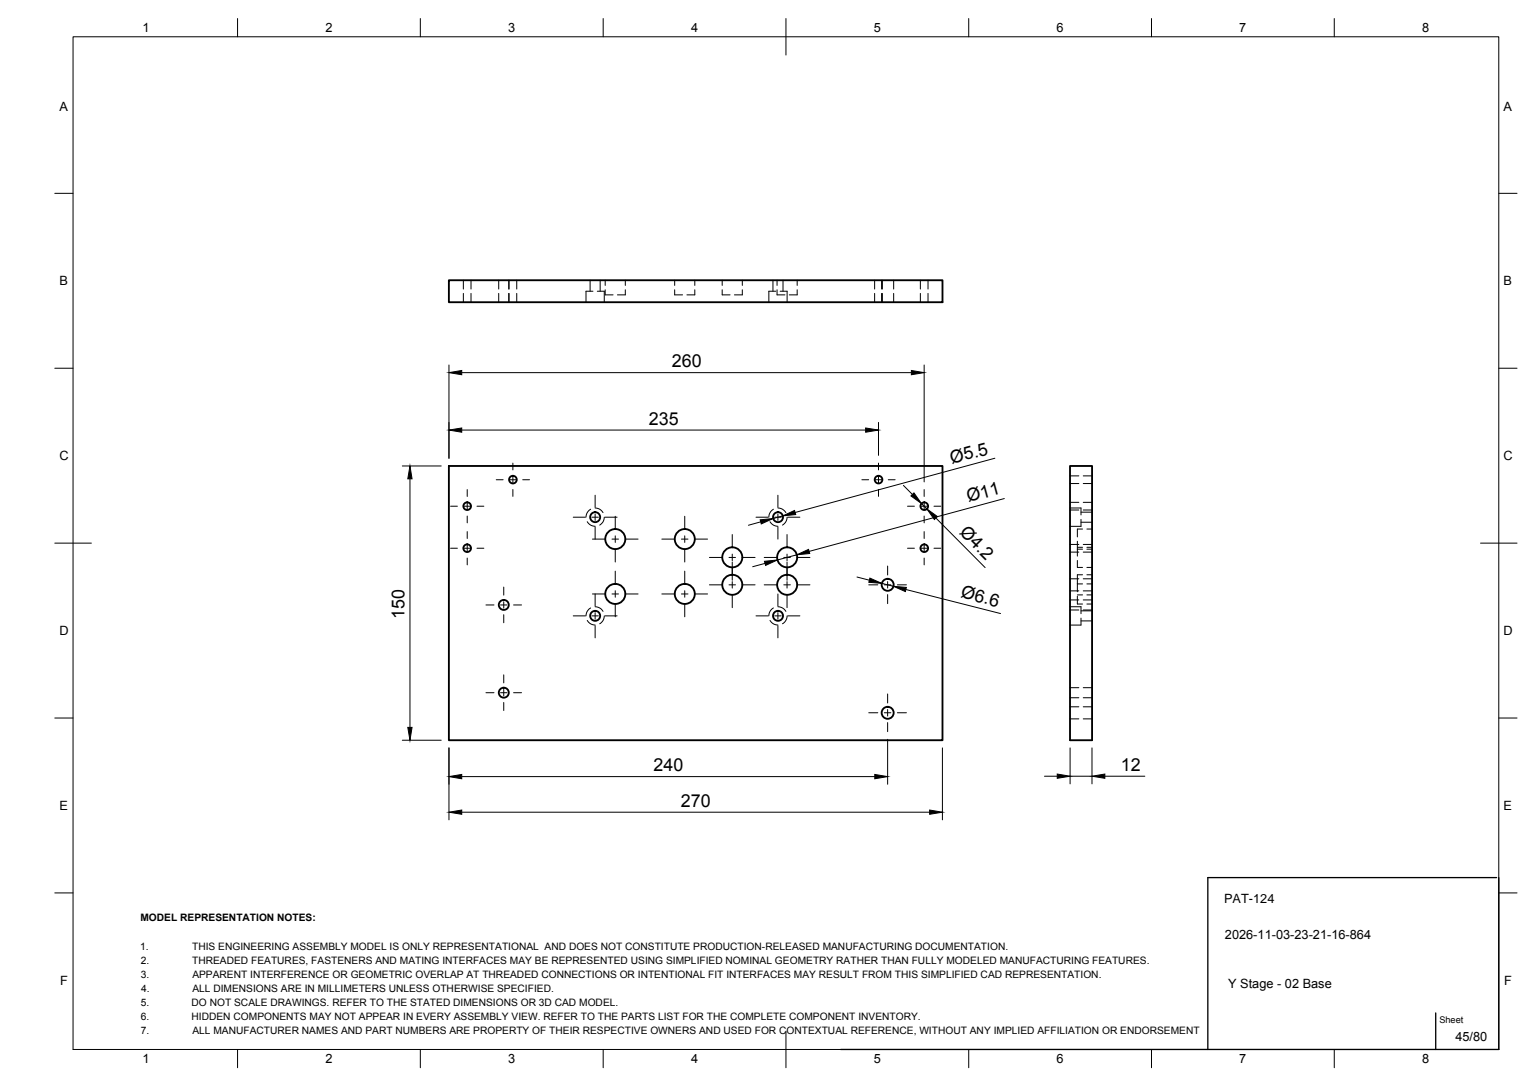
ISO-10303-21;
HEADER;
/* Generated by software containing ST-Developer
 * from STEP Tools, Inc. (www.steptools.com) 
 */

FILE_DESCRIPTION(
/* description */ ('XY cross-slide table'),
/* implementation_level */ '2;1');

FILE_NAME(
/* name */ 'Y Stage - 02 Base.step',
/* time_stamp */ '2026-10-28T03:22:46-07:00',
/* author */ (''),
/* organization */ (''),
/* preprocessor_version */ 'ST-DEVELOPER v20.2',
/* originating_system */ 'Autodesk Translation Framework v15.17.0.0',
/* authorisation */ '');

FILE_SCHEMA (('AUTOMOTIVE_DESIGN { 1 0 10303 214 3 1 1 }'));
ENDSEC;

DATA;
#10=MECHANICAL_DESIGN_GEOMETRIC_PRESENTATION_REPRESENTATION('',(#1727),#62984);
#1546=SHAPE_REPRESENTATION_RELATIONSHIP('SRR','None',#63401,#1629);
#1629=ADVANCED_BREP_SHAPE_REPRESENTATION('',(#1836),#62938);
#1727=STYLED_ITEM('',(#63891),#1836);
#1836=MANIFOLD_SOLID_BREP('Body1',#23025);
#2085=FACE_BOUND('',#5042,.T.);
#2086=FACE_BOUND('',#5045,.T.);
#2087=FACE_BOUND('',#5048,.T.);
#2088=FACE_BOUND('',#5051,.T.);
#2089=FACE_BOUND('',#5071,.T.);
#2090=FACE_BOUND('',#5072,.T.);
#2091=FACE_BOUND('',#5073,.T.);
#2092=FACE_BOUND('',#5074,.T.);
#2093=FACE_BOUND('',#5075,.T.);
#2094=FACE_BOUND('',#5076,.T.);
#2095=FACE_BOUND('',#5077,.T.);
#2096=FACE_BOUND('',#5078,.T.);
#2097=FACE_BOUND('',#5079,.T.);
#2098=FACE_BOUND('',#5080,.T.);
#2099=FACE_BOUND('',#5081,.T.);
#2100=FACE_BOUND('',#5082,.T.);
#2101=FACE_BOUND('',#5083,.T.);
#2102=FACE_BOUND('',#5084,.T.);
#2103=FACE_BOUND('',#5086,.T.);
#2104=FACE_BOUND('',#5087,.T.);
#2105=FACE_BOUND('',#5088,.T.);
#2106=FACE_BOUND('',#5089,.T.);
#2107=FACE_BOUND('',#5090,.T.);
#2108=FACE_BOUND('',#5091,.T.);
#2109=FACE_BOUND('',#5092,.T.);
#2110=FACE_BOUND('',#5093,.T.);
#2111=FACE_BOUND('',#5094,.T.);
#2112=FACE_BOUND('',#5095,.T.);
#2113=FACE_BOUND('',#5096,.T.);
#2114=FACE_BOUND('',#5097,.T.);
#2115=FACE_BOUND('',#5098,.T.);
#2116=FACE_BOUND('',#5099,.T.);
#2117=FACE_BOUND('',#5100,.T.);
#2118=FACE_BOUND('',#5101,.T.);
#2119=FACE_BOUND('',#5102,.T.);
#2120=FACE_BOUND('',#5103,.T.);
#2121=FACE_BOUND('',#5104,.T.);
#2122=FACE_BOUND('',#5105,.T.);
#2123=FACE_BOUND('',#5106,.T.);
#2124=FACE_BOUND('',#5107,.T.);
#2577=PLANE('',#25206);
#2578=PLANE('',#25210);
#2579=PLANE('',#25214);
#2580=PLANE('',#25218);
#2581=PLANE('',#25222);
#2582=PLANE('',#25226);
#2583=PLANE('',#25230);
#2584=PLANE('',#25234);
#2585=PLANE('',#25238);
#2586=PLANE('',#25243);
#2587=PLANE('',#25248);
#2588=PLANE('',#25253);
#2589=PLANE('',#25293);
#2590=PLANE('',#25294);
#2591=PLANE('',#25295);
#2592=PLANE('',#25296);
#2593=PLANE('',#25297);
#2594=PLANE('',#25298);
#3512=FACE_OUTER_BOUND('',#5024,.T.);
#3513=FACE_OUTER_BOUND('',#5025,.T.);
#3514=FACE_OUTER_BOUND('',#5026,.T.);
#3515=FACE_OUTER_BOUND('',#5027,.T.);
#3516=FACE_OUTER_BOUND('',#5028,.T.);
#3517=FACE_OUTER_BOUND('',#5029,.T.);
#3518=FACE_OUTER_BOUND('',#5030,.T.);
#3519=FACE_OUTER_BOUND('',#5031,.T.);
#3520=FACE_OUTER_BOUND('',#5032,.T.);
#3521=FACE_OUTER_BOUND('',#5033,.T.);
#3522=FACE_OUTER_BOUND('',#5034,.T.);
#3523=FACE_OUTER_BOUND('',#5035,.T.);
#3524=FACE_OUTER_BOUND('',#5036,.T.);
#3525=FACE_OUTER_BOUND('',#5037,.T.);
#3526=FACE_OUTER_BOUND('',#5038,.T.);
#3527=FACE_OUTER_BOUND('',#5039,.T.);
#3528=FACE_OUTER_BOUND('',#5040,.T.);
#3529=FACE_OUTER_BOUND('',#5041,.T.);
#3530=FACE_OUTER_BOUND('',#5043,.T.);
#3531=FACE_OUTER_BOUND('',#5044,.T.);
#3532=FACE_OUTER_BOUND('',#5046,.T.);
#3533=FACE_OUTER_BOUND('',#5047,.T.);
#3534=FACE_OUTER_BOUND('',#5049,.T.);
#3535=FACE_OUTER_BOUND('',#5050,.T.);
#3536=FACE_OUTER_BOUND('',#5052,.T.);
#3537=FACE_OUTER_BOUND('',#5053,.T.);
#3538=FACE_OUTER_BOUND('',#5054,.T.);
#3539=FACE_OUTER_BOUND('',#5055,.T.);
#3540=FACE_OUTER_BOUND('',#5056,.T.);
#3541=FACE_OUTER_BOUND('',#5057,.T.);
#3542=FACE_OUTER_BOUND('',#5058,.T.);
#3543=FACE_OUTER_BOUND('',#5059,.T.);
#3544=FACE_OUTER_BOUND('',#5060,.T.);
#3545=FACE_OUTER_BOUND('',#5061,.T.);
#3546=FACE_OUTER_BOUND('',#5062,.T.);
#3547=FACE_OUTER_BOUND('',#5063,.T.);
#3548=FACE_OUTER_BOUND('',#5064,.T.);
#3549=FACE_OUTER_BOUND('',#5065,.T.);
#3550=FACE_OUTER_BOUND('',#5066,.T.);
#3551=FACE_OUTER_BOUND('',#5067,.T.);
#3552=FACE_OUTER_BOUND('',#5068,.T.);
#3553=FACE_OUTER_BOUND('',#5069,.T.);
#3554=FACE_OUTER_BOUND('',#5070,.T.);
#3555=FACE_OUTER_BOUND('',#5085,.T.);
#5024=EDGE_LOOP('',(#17930,#17931,#17932,#17933));
#5025=EDGE_LOOP('',(#17934));
#5026=EDGE_LOOP('',(#17935,#17936,#17937,#17938));
#5027=EDGE_LOOP('',(#17939));
#5028=EDGE_LOOP('',(#17940,#17941,#17942,#17943));
#5029=EDGE_LOOP('',(#17944));
#5030=EDGE_LOOP('',(#17945,#17946,#17947,#17948));
#5031=EDGE_LOOP('',(#17949));
#5032=EDGE_LOOP('',(#17950,#17951,#17952,#17953));
#5033=EDGE_LOOP('',(#17954));
#5034=EDGE_LOOP('',(#17955,#17956,#17957,#17958));
#5035=EDGE_LOOP('',(#17959));
#5036=EDGE_LOOP('',(#17960,#17961,#17962,#17963));
#5037=EDGE_LOOP('',(#17964));
#5038=EDGE_LOOP('',(#17965,#17966,#17967,#17968));
#5039=EDGE_LOOP('',(#17969));
#5040=EDGE_LOOP('',(#17970,#17971,#17972,#17973));
#5041=EDGE_LOOP('',(#17974));
#5042=EDGE_LOOP('',(#17975));
#5043=EDGE_LOOP('',(#17976,#17977,#17978,#17979));
#5044=EDGE_LOOP('',(#17980));
#5045=EDGE_LOOP('',(#17981));
#5046=EDGE_LOOP('',(#17982,#17983,#17984,#17985));
#5047=EDGE_LOOP('',(#17986));
#5048=EDGE_LOOP('',(#17987));
#5049=EDGE_LOOP('',(#17988,#17989,#17990,#17991));
#5050=EDGE_LOOP('',(#17992));
#5051=EDGE_LOOP('',(#17993));
#5052=EDGE_LOOP('',(#17994,#17995,#17996,#17997));
#5053=EDGE_LOOP('',(#17998,#17999,#18000,#18001));
#5054=EDGE_LOOP('',(#18002,#18003,#18004,#18005));
#5055=EDGE_LOOP('',(#18006,#18007,#18008,#18009));
#5056=EDGE_LOOP('',(#18010,#18011,#18012,#18013));
#5057=EDGE_LOOP('',(#18014,#18015,#18016,#18017));
#5058=EDGE_LOOP('',(#18018,#18019,#18020,#18021));
#5059=EDGE_LOOP('',(#18022,#18023,#18024,#18025));
#5060=EDGE_LOOP('',(#18026,#18027,#18028,#18029));
#5061=EDGE_LOOP('',(#18030,#18031,#18032,#18033));
#5062=EDGE_LOOP('',(#18034,#18035,#18036,#18037));
#5063=EDGE_LOOP('',(#18038,#18039,#18040,#18041));
#5064=EDGE_LOOP('',(#18042,#18043,#18044,#18045));
#5065=EDGE_LOOP('',(#18046,#18047,#18048,#18049));
#5066=EDGE_LOOP('',(#18050,#18051,#18052,#18053));
#5067=EDGE_LOOP('',(#18054,#18055,#18056,#18057));
#5068=EDGE_LOOP('',(#18058,#18059,#18060,#18061));
#5069=EDGE_LOOP('',(#18062,#18063,#18064,#18065));
#5070=EDGE_LOOP('',(#18066,#18067,#18068,#18069));
#5071=EDGE_LOOP('',(#18070));
#5072=EDGE_LOOP('',(#18071));
#5073=EDGE_LOOP('',(#18072));
#5074=EDGE_LOOP('',(#18073));
#5075=EDGE_LOOP('',(#18074));
#5076=EDGE_LOOP('',(#18075));
#5077=EDGE_LOOP('',(#18076));
#5078=EDGE_LOOP('',(#18077));
#5079=EDGE_LOOP('',(#18078));
#5080=EDGE_LOOP('',(#18079));
#5081=EDGE_LOOP('',(#18080));
#5082=EDGE_LOOP('',(#18081));
#5083=EDGE_LOOP('',(#18082));
#5084=EDGE_LOOP('',(#18083));
#5085=EDGE_LOOP('',(#18084,#18085,#18086,#18087));
#5086=EDGE_LOOP('',(#18088));
#5087=EDGE_LOOP('',(#18089));
#5088=EDGE_LOOP('',(#18090));
#5089=EDGE_LOOP('',(#18091));
#5090=EDGE_LOOP('',(#18092));
#5091=EDGE_LOOP('',(#18093));
#5092=EDGE_LOOP('',(#18094));
#5093=EDGE_LOOP('',(#18095));
#5094=EDGE_LOOP('',(#18096));
#5095=EDGE_LOOP('',(#18097));
#5096=EDGE_LOOP('',(#18098));
#5097=EDGE_LOOP('',(#18099));
#5098=EDGE_LOOP('',(#18100));
#5099=EDGE_LOOP('',(#18101));
#5100=EDGE_LOOP('',(#18102));
#5101=EDGE_LOOP('',(#18103));
#5102=EDGE_LOOP('',(#18104));
#5103=EDGE_LOOP('',(#18105));
#5104=EDGE_LOOP('',(#18106));
#5105=EDGE_LOOP('',(#18107));
#5106=EDGE_LOOP('',(#18108));
#5107=EDGE_LOOP('',(#18109));
#6644=LINE('',#47786,#8131);
#6645=LINE('',#47793,#8132);
#6646=LINE('',#47800,#8133);
#6647=LINE('',#47807,#8134);
#6648=LINE('',#47814,#8135);
#6649=LINE('',#47821,#8136);
#6650=LINE('',#47828,#8137);
#6651=LINE('',#47835,#8138);
#6652=LINE('',#47842,#8139);
#6653=LINE('',#47851,#8140);
#6654=LINE('',#47860,#8141);
#6655=LINE('',#47869,#8142);
#6656=LINE('',#47877,#8143);
#6657=LINE('',#47881,#8144);
#6658=LINE('',#47885,#8145);
#6659=LINE('',#47889,#8146);
#6660=LINE('',#47894,#8147);
#6661=LINE('',#47900,#8148);
#6662=LINE('',#47906,#8149);
#6663=LINE('',#47912,#8150);
#6664=LINE('',#47918,#8151);
#6665=LINE('',#47924,#8152);
#6666=LINE('',#47930,#8153);
#6667=LINE('',#47936,#8154);
#6668=LINE('',#47942,#8155);
#6669=LINE('',#47948,#8156);
#6670=LINE('',#47953,#8157);
#6671=LINE('',#47955,#8158);
#6672=LINE('',#47957,#8159);
#6673=LINE('',#47958,#8160);
#6674=LINE('',#47961,#8161);
#6675=LINE('',#47963,#8162);
#6676=LINE('',#47964,#8163);
#6677=LINE('',#47967,#8164);
#6678=LINE('',#47969,#8165);
#6679=LINE('',#47970,#8166);
#6680=LINE('',#47972,#8167);
#6681=LINE('',#47973,#8168);
#8131=VECTOR('',#29609,0.550000000000001);
#8132=VECTOR('',#29618,0.550000000000001);
#8133=VECTOR('',#29627,0.550000000000001);
#8134=VECTOR('',#29636,0.550000000000001);
#8135=VECTOR('',#29645,0.550000000000001);
#8136=VECTOR('',#29654,0.550000000000001);
#8137=VECTOR('',#29663,0.550000000000001);
#8138=VECTOR('',#29672,0.550000000000001);
#8139=VECTOR('',#29681,0.5);
#8140=VECTOR('',#29692,0.5);
#8141=VECTOR('',#29703,0.5);
#8142=VECTOR('',#29714,0.5);
#8143=VECTOR('',#29725,0.275);
#8144=VECTOR('',#29730,0.274999999999999);
#8145=VECTOR('',#29735,0.275);
#8146=VECTOR('',#29740,0.274999999999999);
#8147=VECTOR('',#29745,0.210000000000001);
#8148=VECTOR('',#29752,0.21);
#8149=VECTOR('',#29759,0.329999999999998);
#8150=VECTOR('',#29766,0.329999999999998);
#8151=VECTOR('',#29773,0.275);
#8152=VECTOR('',#29780,0.275);
#8153=VECTOR('',#29787,0.210000000000001);
#8154=VECTOR('',#29794,0.21);
#8155=VECTOR('',#29801,0.21);
#8156=VECTOR('',#29808,0.210000000000001);
#8157=VECTOR('',#29813,1.);
#8158=VECTOR('',#29814,1.);
#8159=VECTOR('',#29815,1.);
#8160=VECTOR('',#29816,1.);
#8161=VECTOR('',#29819,1.);
#8162=VECTOR('',#29820,1.);
#8163=VECTOR('',#29821,1.);
#8164=VECTOR('',#29824,1.);
#8165=VECTOR('',#29825,1.);
#8166=VECTOR('',#29826,1.);
#8167=VECTOR('',#29829,1.);
#8168=VECTOR('',#29830,1.);
#9311=CIRCLE('',#25204,0.550000000000001);
#9312=CIRCLE('',#25205,0.550000000000001);
#9313=CIRCLE('',#25208,0.550000000000001);
#9314=CIRCLE('',#25209,0.550000000000001);
#9315=CIRCLE('',#25212,0.550000000000001);
#9316=CIRCLE('',#25213,0.550000000000001);
#9317=CIRCLE('',#25216,0.550000000000001);
#9318=CIRCLE('',#25217,0.550000000000001);
#9319=CIRCLE('',#25220,0.550000000000001);
#9320=CIRCLE('',#25221,0.550000000000001);
#9321=CIRCLE('',#25224,0.550000000000001);
#9322=CIRCLE('',#25225,0.550000000000001);
#9323=CIRCLE('',#25228,0.550000000000001);
#9324=CIRCLE('',#25229,0.550000000000001);
#9325=CIRCLE('',#25232,0.550000000000001);
#9326=CIRCLE('',#25233,0.550000000000001);
#9327=CIRCLE('',#25236,0.5);
#9328=CIRCLE('',#25237,0.5);
#9329=CIRCLE('',#25239,0.275);
#9330=CIRCLE('',#25241,0.5);
#9331=CIRCLE('',#25242,0.5);
#9332=CIRCLE('',#25244,0.274999999999999);
#9333=CIRCLE('',#25246,0.5);
#9334=CIRCLE('',#25247,0.5);
#9335=CIRCLE('',#25249,0.275);
#9336=CIRCLE('',#25251,0.5);
#9337=CIRCLE('',#25252,0.5);
#9338=CIRCLE('',#25254,0.274999999999999);
#9339=CIRCLE('',#25256,0.275);
#9340=CIRCLE('',#25258,0.274999999999999);
#9341=CIRCLE('',#25260,0.275);
#9342=CIRCLE('',#25262,0.274999999999999);
#9343=CIRCLE('',#25264,0.210000000000001);
#9344=CIRCLE('',#25265,0.210000000000001);
#9345=CIRCLE('',#25267,0.21);
#9346=CIRCLE('',#25268,0.21);
#9347=CIRCLE('',#25270,0.329999999999998);
#9348=CIRCLE('',#25271,0.329999999999998);
#9349=CIRCLE('',#25273,0.329999999999998);
#9350=CIRCLE('',#25274,0.329999999999998);
#9351=CIRCLE('',#25276,0.275);
#9352=CIRCLE('',#25277,0.275);
#9353=CIRCLE('',#25279,0.275);
#9354=CIRCLE('',#25280,0.275);
#9355=CIRCLE('',#25282,0.210000000000001);
#9356=CIRCLE('',#25283,0.210000000000001);
#9357=CIRCLE('',#25285,0.21);
#9358=CIRCLE('',#25286,0.21);
#9359=CIRCLE('',#25288,0.21);
#9360=CIRCLE('',#25289,0.21);
#9361=CIRCLE('',#25291,0.210000000000001);
#9362=CIRCLE('',#25292,0.210000000000001);
#10791=VERTEX_POINT('',#47783);
#10792=VERTEX_POINT('',#47785);
#10793=VERTEX_POINT('',#47790);
#10794=VERTEX_POINT('',#47792);
#10795=VERTEX_POINT('',#47797);
#10796=VERTEX_POINT('',#47799);
#10797=VERTEX_POINT('',#47804);
#10798=VERTEX_POINT('',#47806);
#10799=VERTEX_POINT('',#47811);
#10800=VERTEX_POINT('',#47813);
#10801=VERTEX_POINT('',#47818);
#10802=VERTEX_POINT('',#47820);
#10803=VERTEX_POINT('',#47825);
#10804=VERTEX_POINT('',#47827);
#10805=VERTEX_POINT('',#47832);
#10806=VERTEX_POINT('',#47834);
#10807=VERTEX_POINT('',#47839);
#10808=VERTEX_POINT('',#47841);
#10809=VERTEX_POINT('',#47845);
#10810=VERTEX_POINT('',#47848);
#10811=VERTEX_POINT('',#47850);
#10812=VERTEX_POINT('',#47854);
#10813=VERTEX_POINT('',#47857);
#10814=VERTEX_POINT('',#47859);
#10815=VERTEX_POINT('',#47863);
#10816=VERTEX_POINT('',#47866);
#10817=VERTEX_POINT('',#47868);
#10818=VERTEX_POINT('',#47872);
#10819=VERTEX_POINT('',#47875);
#10820=VERTEX_POINT('',#47879);
#10821=VERTEX_POINT('',#47883);
#10822=VERTEX_POINT('',#47887);
#10823=VERTEX_POINT('',#47891);
#10824=VERTEX_POINT('',#47893);
#10825=VERTEX_POINT('',#47897);
#10826=VERTEX_POINT('',#47899);
#10827=VERTEX_POINT('',#47903);
#10828=VERTEX_POINT('',#47905);
#10829=VERTEX_POINT('',#47909);
#10830=VERTEX_POINT('',#47911);
#10831=VERTEX_POINT('',#47915);
#10832=VERTEX_POINT('',#47917);
#10833=VERTEX_POINT('',#47921);
#10834=VERTEX_POINT('',#47923);
#10835=VERTEX_POINT('',#47927);
#10836=VERTEX_POINT('',#47929);
#10837=VERTEX_POINT('',#47933);
#10838=VERTEX_POINT('',#47935);
#10839=VERTEX_POINT('',#47939);
#10840=VERTEX_POINT('',#47941);
#10841=VERTEX_POINT('',#47945);
#10842=VERTEX_POINT('',#47947);
#10843=VERTEX_POINT('',#47951);
#10844=VERTEX_POINT('',#47952);
#10845=VERTEX_POINT('',#47954);
#10846=VERTEX_POINT('',#47956);
#10847=VERTEX_POINT('',#47960);
#10848=VERTEX_POINT('',#47962);
#10849=VERTEX_POINT('',#47966);
#10850=VERTEX_POINT('',#47968);
#13349=EDGE_CURVE('',#10791,#10791,#9311,.T.);
#13350=EDGE_CURVE('',#10791,#10792,#6644,.T.);
#13351=EDGE_CURVE('',#10792,#10792,#9312,.T.);
#13352=EDGE_CURVE('',#10793,#10793,#9313,.T.);
#13353=EDGE_CURVE('',#10793,#10794,#6645,.T.);
#13354=EDGE_CURVE('',#10794,#10794,#9314,.T.);
#13355=EDGE_CURVE('',#10795,#10795,#9315,.T.);
#13356=EDGE_CURVE('',#10795,#10796,#6646,.T.);
#13357=EDGE_CURVE('',#10796,#10796,#9316,.T.);
#13358=EDGE_CURVE('',#10797,#10797,#9317,.T.);
#13359=EDGE_CURVE('',#10797,#10798,#6647,.T.);
#13360=EDGE_CURVE('',#10798,#10798,#9318,.T.);
#13361=EDGE_CURVE('',#10799,#10799,#9319,.T.);
#13362=EDGE_CURVE('',#10799,#10800,#6648,.T.);
#13363=EDGE_CURVE('',#10800,#10800,#9320,.T.);
#13364=EDGE_CURVE('',#10801,#10801,#9321,.T.);
#13365=EDGE_CURVE('',#10801,#10802,#6649,.T.);
#13366=EDGE_CURVE('',#10802,#10802,#9322,.T.);
#13367=EDGE_CURVE('',#10803,#10803,#9323,.T.);
#13368=EDGE_CURVE('',#10803,#10804,#6650,.T.);
#13369=EDGE_CURVE('',#10804,#10804,#9324,.T.);
#13370=EDGE_CURVE('',#10805,#10805,#9325,.T.);
#13371=EDGE_CURVE('',#10805,#10806,#6651,.T.);
#13372=EDGE_CURVE('',#10806,#10806,#9326,.T.);
#13373=EDGE_CURVE('',#10807,#10807,#9327,.T.);
#13374=EDGE_CURVE('',#10807,#10808,#6652,.T.);
#13375=EDGE_CURVE('',#10808,#10808,#9328,.T.);
#13376=EDGE_CURVE('',#10809,#10809,#9329,.T.);
#13377=EDGE_CURVE('',#10810,#10810,#9330,.T.);
#13378=EDGE_CURVE('',#10810,#10811,#6653,.T.);
#13379=EDGE_CURVE('',#10811,#10811,#9331,.T.);
#13380=EDGE_CURVE('',#10812,#10812,#9332,.T.);
#13381=EDGE_CURVE('',#10813,#10813,#9333,.T.);
#13382=EDGE_CURVE('',#10813,#10814,#6654,.T.);
#13383=EDGE_CURVE('',#10814,#10814,#9334,.T.);
#13384=EDGE_CURVE('',#10815,#10815,#9335,.T.);
#13385=EDGE_CURVE('',#10816,#10816,#9336,.T.);
#13386=EDGE_CURVE('',#10816,#10817,#6655,.T.);
#13387=EDGE_CURVE('',#10817,#10817,#9337,.T.);
#13388=EDGE_CURVE('',#10818,#10818,#9338,.T.);
#13389=EDGE_CURVE('',#10819,#10819,#9339,.T.);
#13390=EDGE_CURVE('',#10819,#10809,#6656,.T.);
#13391=EDGE_CURVE('',#10820,#10820,#9340,.T.);
#13392=EDGE_CURVE('',#10820,#10812,#6657,.T.);
#13393=EDGE_CURVE('',#10821,#10821,#9341,.T.);
#13394=EDGE_CURVE('',#10821,#10815,#6658,.T.);
#13395=EDGE_CURVE('',#10822,#10822,#9342,.T.);
#13396=EDGE_CURVE('',#10822,#10818,#6659,.T.);
#13397=EDGE_CURVE('',#10823,#10823,#9343,.T.);
#13398=EDGE_CURVE('',#10823,#10824,#6660,.T.);
#13399=EDGE_CURVE('',#10824,#10824,#9344,.T.);
#13400=EDGE_CURVE('',#10825,#10825,#9345,.T.);
#13401=EDGE_CURVE('',#10825,#10826,#6661,.T.);
#13402=EDGE_CURVE('',#10826,#10826,#9346,.T.);
#13403=EDGE_CURVE('',#10827,#10827,#9347,.T.);
#13404=EDGE_CURVE('',#10827,#10828,#6662,.T.);
#13405=EDGE_CURVE('',#10828,#10828,#9348,.T.);
#13406=EDGE_CURVE('',#10829,#10829,#9349,.T.);
#13407=EDGE_CURVE('',#10829,#10830,#6663,.T.);
#13408=EDGE_CURVE('',#10830,#10830,#9350,.T.);
#13409=EDGE_CURVE('',#10831,#10831,#9351,.T.);
#13410=EDGE_CURVE('',#10831,#10832,#6664,.T.);
#13411=EDGE_CURVE('',#10832,#10832,#9352,.T.);
#13412=EDGE_CURVE('',#10833,#10833,#9353,.T.);
#13413=EDGE_CURVE('',#10833,#10834,#6665,.T.);
#13414=EDGE_CURVE('',#10834,#10834,#9354,.T.);
#13415=EDGE_CURVE('',#10835,#10835,#9355,.T.);
#13416=EDGE_CURVE('',#10835,#10836,#6666,.T.);
#13417=EDGE_CURVE('',#10836,#10836,#9356,.T.);
#13418=EDGE_CURVE('',#10837,#10837,#9357,.T.);
#13419=EDGE_CURVE('',#10837,#10838,#6667,.T.);
#13420=EDGE_CURVE('',#10838,#10838,#9358,.T.);
#13421=EDGE_CURVE('',#10839,#10839,#9359,.T.);
#13422=EDGE_CURVE('',#10839,#10840,#6668,.T.);
#13423=EDGE_CURVE('',#10840,#10840,#9360,.T.);
#13424=EDGE_CURVE('',#10841,#10841,#9361,.T.);
#13425=EDGE_CURVE('',#10841,#10842,#6669,.T.);
#13426=EDGE_CURVE('',#10842,#10842,#9362,.T.);
#13427=EDGE_CURVE('',#10843,#10844,#6670,.T.);
#13428=EDGE_CURVE('',#10844,#10845,#6671,.T.);
#13429=EDGE_CURVE('',#10846,#10845,#6672,.T.);
#13430=EDGE_CURVE('',#10843,#10846,#6673,.T.);
#13431=EDGE_CURVE('',#10847,#10843,#6674,.T.);
#13432=EDGE_CURVE('',#10848,#10846,#6675,.T.);
#13433=EDGE_CURVE('',#10847,#10848,#6676,.T.);
#13434=EDGE_CURVE('',#10849,#10847,#6677,.T.);
#13435=EDGE_CURVE('',#10850,#10848,#6678,.T.);
#13436=EDGE_CURVE('',#10849,#10850,#6679,.T.);
#13437=EDGE_CURVE('',#10844,#10849,#6680,.T.);
#13438=EDGE_CURVE('',#10845,#10850,#6681,.T.);
#17930=ORIENTED_EDGE('',*,*,#13349,.F.);
#17931=ORIENTED_EDGE('',*,*,#13350,.T.);
#17932=ORIENTED_EDGE('',*,*,#13351,.T.);
#17933=ORIENTED_EDGE('',*,*,#13350,.F.);
#17934=ORIENTED_EDGE('',*,*,#13351,.F.);
#17935=ORIENTED_EDGE('',*,*,#13352,.F.);
#17936=ORIENTED_EDGE('',*,*,#13353,.T.);
#17937=ORIENTED_EDGE('',*,*,#13354,.T.);
#17938=ORIENTED_EDGE('',*,*,#13353,.F.);
#17939=ORIENTED_EDGE('',*,*,#13354,.F.);
#17940=ORIENTED_EDGE('',*,*,#13355,.F.);
#17941=ORIENTED_EDGE('',*,*,#13356,.T.);
#17942=ORIENTED_EDGE('',*,*,#13357,.T.);
#17943=ORIENTED_EDGE('',*,*,#13356,.F.);
#17944=ORIENTED_EDGE('',*,*,#13357,.F.);
#17945=ORIENTED_EDGE('',*,*,#13358,.F.);
#17946=ORIENTED_EDGE('',*,*,#13359,.T.);
#17947=ORIENTED_EDGE('',*,*,#13360,.T.);
#17948=ORIENTED_EDGE('',*,*,#13359,.F.);
#17949=ORIENTED_EDGE('',*,*,#13360,.F.);
#17950=ORIENTED_EDGE('',*,*,#13361,.F.);
#17951=ORIENTED_EDGE('',*,*,#13362,.T.);
#17952=ORIENTED_EDGE('',*,*,#13363,.T.);
#17953=ORIENTED_EDGE('',*,*,#13362,.F.);
#17954=ORIENTED_EDGE('',*,*,#13363,.F.);
#17955=ORIENTED_EDGE('',*,*,#13364,.F.);
#17956=ORIENTED_EDGE('',*,*,#13365,.T.);
#17957=ORIENTED_EDGE('',*,*,#13366,.T.);
#17958=ORIENTED_EDGE('',*,*,#13365,.F.);
#17959=ORIENTED_EDGE('',*,*,#13366,.F.);
#17960=ORIENTED_EDGE('',*,*,#13367,.F.);
#17961=ORIENTED_EDGE('',*,*,#13368,.T.);
#17962=ORIENTED_EDGE('',*,*,#13369,.T.);
#17963=ORIENTED_EDGE('',*,*,#13368,.F.);
#17964=ORIENTED_EDGE('',*,*,#13369,.F.);
#17965=ORIENTED_EDGE('',*,*,#13370,.F.);
#17966=ORIENTED_EDGE('',*,*,#13371,.T.);
#17967=ORIENTED_EDGE('',*,*,#13372,.T.);
#17968=ORIENTED_EDGE('',*,*,#13371,.F.);
#17969=ORIENTED_EDGE('',*,*,#13372,.F.);
#17970=ORIENTED_EDGE('',*,*,#13373,.F.);
#17971=ORIENTED_EDGE('',*,*,#13374,.T.);
#17972=ORIENTED_EDGE('',*,*,#13375,.F.);
#17973=ORIENTED_EDGE('',*,*,#13374,.F.);
#17974=ORIENTED_EDGE('',*,*,#13373,.T.);
#17975=ORIENTED_EDGE('',*,*,#13376,.F.);
#17976=ORIENTED_EDGE('',*,*,#13377,.F.);
#17977=ORIENTED_EDGE('',*,*,#13378,.T.);
#17978=ORIENTED_EDGE('',*,*,#13379,.F.);
#17979=ORIENTED_EDGE('',*,*,#13378,.F.);
#17980=ORIENTED_EDGE('',*,*,#13377,.T.);
#17981=ORIENTED_EDGE('',*,*,#13380,.F.);
#17982=ORIENTED_EDGE('',*,*,#13381,.F.);
#17983=ORIENTED_EDGE('',*,*,#13382,.T.);
#17984=ORIENTED_EDGE('',*,*,#13383,.F.);
#17985=ORIENTED_EDGE('',*,*,#13382,.F.);
#17986=ORIENTED_EDGE('',*,*,#13381,.T.);
#17987=ORIENTED_EDGE('',*,*,#13384,.F.);
#17988=ORIENTED_EDGE('',*,*,#13385,.F.);
#17989=ORIENTED_EDGE('',*,*,#13386,.T.);
#17990=ORIENTED_EDGE('',*,*,#13387,.F.);
#17991=ORIENTED_EDGE('',*,*,#13386,.F.);
#17992=ORIENTED_EDGE('',*,*,#13385,.T.);
#17993=ORIENTED_EDGE('',*,*,#13388,.F.);
#17994=ORIENTED_EDGE('',*,*,#13389,.F.);
#17995=ORIENTED_EDGE('',*,*,#13390,.T.);
#17996=ORIENTED_EDGE('',*,*,#13376,.T.);
#17997=ORIENTED_EDGE('',*,*,#13390,.F.);
#17998=ORIENTED_EDGE('',*,*,#13391,.F.);
#17999=ORIENTED_EDGE('',*,*,#13392,.T.);
#18000=ORIENTED_EDGE('',*,*,#13380,.T.);
#18001=ORIENTED_EDGE('',*,*,#13392,.F.);
#18002=ORIENTED_EDGE('',*,*,#13393,.F.);
#18003=ORIENTED_EDGE('',*,*,#13394,.T.);
#18004=ORIENTED_EDGE('',*,*,#13384,.T.);
#18005=ORIENTED_EDGE('',*,*,#13394,.F.);
#18006=ORIENTED_EDGE('',*,*,#13395,.F.);
#18007=ORIENTED_EDGE('',*,*,#13396,.T.);
#18008=ORIENTED_EDGE('',*,*,#13388,.T.);
#18009=ORIENTED_EDGE('',*,*,#13396,.F.);
#18010=ORIENTED_EDGE('',*,*,#13397,.F.);
#18011=ORIENTED_EDGE('',*,*,#13398,.T.);
#18012=ORIENTED_EDGE('',*,*,#13399,.F.);
#18013=ORIENTED_EDGE('',*,*,#13398,.F.);
#18014=ORIENTED_EDGE('',*,*,#13400,.F.);
#18015=ORIENTED_EDGE('',*,*,#13401,.T.);
#18016=ORIENTED_EDGE('',*,*,#13402,.F.);
#18017=ORIENTED_EDGE('',*,*,#13401,.F.);
#18018=ORIENTED_EDGE('',*,*,#13403,.F.);
#18019=ORIENTED_EDGE('',*,*,#13404,.T.);
#18020=ORIENTED_EDGE('',*,*,#13405,.F.);
#18021=ORIENTED_EDGE('',*,*,#13404,.F.);
#18022=ORIENTED_EDGE('',*,*,#13406,.F.);
#18023=ORIENTED_EDGE('',*,*,#13407,.T.);
#18024=ORIENTED_EDGE('',*,*,#13408,.F.);
#18025=ORIENTED_EDGE('',*,*,#13407,.F.);
#18026=ORIENTED_EDGE('',*,*,#13409,.F.);
#18027=ORIENTED_EDGE('',*,*,#13410,.T.);
#18028=ORIENTED_EDGE('',*,*,#13411,.F.);
#18029=ORIENTED_EDGE('',*,*,#13410,.F.);
#18030=ORIENTED_EDGE('',*,*,#13412,.F.);
#18031=ORIENTED_EDGE('',*,*,#13413,.T.);
#18032=ORIENTED_EDGE('',*,*,#13414,.F.);
#18033=ORIENTED_EDGE('',*,*,#13413,.F.);
#18034=ORIENTED_EDGE('',*,*,#13415,.F.);
#18035=ORIENTED_EDGE('',*,*,#13416,.T.);
#18036=ORIENTED_EDGE('',*,*,#13417,.F.);
#18037=ORIENTED_EDGE('',*,*,#13416,.F.);
#18038=ORIENTED_EDGE('',*,*,#13418,.F.);
#18039=ORIENTED_EDGE('',*,*,#13419,.T.);
#18040=ORIENTED_EDGE('',*,*,#13420,.F.);
#18041=ORIENTED_EDGE('',*,*,#13419,.F.);
#18042=ORIENTED_EDGE('',*,*,#13421,.F.);
#18043=ORIENTED_EDGE('',*,*,#13422,.T.);
#18044=ORIENTED_EDGE('',*,*,#13423,.F.);
#18045=ORIENTED_EDGE('',*,*,#13422,.F.);
#18046=ORIENTED_EDGE('',*,*,#13424,.F.);
#18047=ORIENTED_EDGE('',*,*,#13425,.T.);
#18048=ORIENTED_EDGE('',*,*,#13426,.F.);
#18049=ORIENTED_EDGE('',*,*,#13425,.F.);
#18050=ORIENTED_EDGE('',*,*,#13427,.T.);
#18051=ORIENTED_EDGE('',*,*,#13428,.T.);
#18052=ORIENTED_EDGE('',*,*,#13429,.F.);
#18053=ORIENTED_EDGE('',*,*,#13430,.F.);
#18054=ORIENTED_EDGE('',*,*,#13431,.T.);
#18055=ORIENTED_EDGE('',*,*,#13430,.T.);
#18056=ORIENTED_EDGE('',*,*,#13432,.F.);
#18057=ORIENTED_EDGE('',*,*,#13433,.F.);
#18058=ORIENTED_EDGE('',*,*,#13434,.T.);
#18059=ORIENTED_EDGE('',*,*,#13433,.T.);
#18060=ORIENTED_EDGE('',*,*,#13435,.F.);
#18061=ORIENTED_EDGE('',*,*,#13436,.F.);
#18062=ORIENTED_EDGE('',*,*,#13437,.T.);
#18063=ORIENTED_EDGE('',*,*,#13436,.T.);
#18064=ORIENTED_EDGE('',*,*,#13438,.F.);
#18065=ORIENTED_EDGE('',*,*,#13428,.F.);
#18066=ORIENTED_EDGE('',*,*,#13438,.T.);
#18067=ORIENTED_EDGE('',*,*,#13435,.T.);
#18068=ORIENTED_EDGE('',*,*,#13432,.T.);
#18069=ORIENTED_EDGE('',*,*,#13429,.T.);
#18070=ORIENTED_EDGE('',*,*,#13402,.T.);
#18071=ORIENTED_EDGE('',*,*,#13426,.T.);
#18072=ORIENTED_EDGE('',*,*,#13423,.T.);
#18073=ORIENTED_EDGE('',*,*,#13420,.T.);
#18074=ORIENTED_EDGE('',*,*,#13417,.T.);
#18075=ORIENTED_EDGE('',*,*,#13414,.T.);
#18076=ORIENTED_EDGE('',*,*,#13411,.T.);
#18077=ORIENTED_EDGE('',*,*,#13408,.T.);
#18078=ORIENTED_EDGE('',*,*,#13405,.T.);
#18079=ORIENTED_EDGE('',*,*,#13399,.T.);
#18080=ORIENTED_EDGE('',*,*,#13387,.T.);
#18081=ORIENTED_EDGE('',*,*,#13383,.T.);
#18082=ORIENTED_EDGE('',*,*,#13379,.T.);
#18083=ORIENTED_EDGE('',*,*,#13375,.T.);
#18084=ORIENTED_EDGE('',*,*,#13437,.F.);
#18085=ORIENTED_EDGE('',*,*,#13427,.F.);
#18086=ORIENTED_EDGE('',*,*,#13431,.F.);
#18087=ORIENTED_EDGE('',*,*,#13434,.F.);
#18088=ORIENTED_EDGE('',*,*,#13389,.T.);
#18089=ORIENTED_EDGE('',*,*,#13391,.T.);
#18090=ORIENTED_EDGE('',*,*,#13393,.T.);
#18091=ORIENTED_EDGE('',*,*,#13395,.T.);
#18092=ORIENTED_EDGE('',*,*,#13400,.T.);
#18093=ORIENTED_EDGE('',*,*,#13424,.T.);
#18094=ORIENTED_EDGE('',*,*,#13421,.T.);
#18095=ORIENTED_EDGE('',*,*,#13418,.T.);
#18096=ORIENTED_EDGE('',*,*,#13415,.T.);
#18097=ORIENTED_EDGE('',*,*,#13412,.T.);
#18098=ORIENTED_EDGE('',*,*,#13409,.T.);
#18099=ORIENTED_EDGE('',*,*,#13406,.T.);
#18100=ORIENTED_EDGE('',*,*,#13403,.T.);
#18101=ORIENTED_EDGE('',*,*,#13397,.T.);
#18102=ORIENTED_EDGE('',*,*,#13370,.T.);
#18103=ORIENTED_EDGE('',*,*,#13367,.T.);
#18104=ORIENTED_EDGE('',*,*,#13364,.T.);
#18105=ORIENTED_EDGE('',*,*,#13361,.T.);
#18106=ORIENTED_EDGE('',*,*,#13358,.T.);
#18107=ORIENTED_EDGE('',*,*,#13355,.T.);
#18108=ORIENTED_EDGE('',*,*,#13352,.T.);
#18109=ORIENTED_EDGE('',*,*,#13349,.T.);
#21338=CYLINDRICAL_SURFACE('',#25203,0.550000000000001);
#21339=CYLINDRICAL_SURFACE('',#25207,0.550000000000001);
#21340=CYLINDRICAL_SURFACE('',#25211,0.550000000000001);
#21341=CYLINDRICAL_SURFACE('',#25215,0.550000000000001);
#21342=CYLINDRICAL_SURFACE('',#25219,0.550000000000001);
#21343=CYLINDRICAL_SURFACE('',#25223,0.550000000000001);
#21344=CYLINDRICAL_SURFACE('',#25227,0.550000000000001);
#21345=CYLINDRICAL_SURFACE('',#25231,0.550000000000001);
#21346=CYLINDRICAL_SURFACE('',#25235,0.5);
#21347=CYLINDRICAL_SURFACE('',#25240,0.5);
#21348=CYLINDRICAL_SURFACE('',#25245,0.5);
#21349=CYLINDRICAL_SURFACE('',#25250,0.5);
#21350=CYLINDRICAL_SURFACE('',#25255,0.275);
#21351=CYLINDRICAL_SURFACE('',#25257,0.274999999999999);
#21352=CYLINDRICAL_SURFACE('',#25259,0.275);
#21353=CYLINDRICAL_SURFACE('',#25261,0.274999999999999);
#21354=CYLINDRICAL_SURFACE('',#25263,0.210000000000001);
#21355=CYLINDRICAL_SURFACE('',#25266,0.21);
#21356=CYLINDRICAL_SURFACE('',#25269,0.329999999999998);
#21357=CYLINDRICAL_SURFACE('',#25272,0.329999999999998);
#21358=CYLINDRICAL_SURFACE('',#25275,0.275);
#21359=CYLINDRICAL_SURFACE('',#25278,0.275);
#21360=CYLINDRICAL_SURFACE('',#25281,0.210000000000001);
#21361=CYLINDRICAL_SURFACE('',#25284,0.21);
#21362=CYLINDRICAL_SURFACE('',#25287,0.21);
#21363=CYLINDRICAL_SURFACE('',#25290,0.210000000000001);
#22293=ADVANCED_FACE('',(#3512),#21338,.F.);
#22294=ADVANCED_FACE('',(#3513),#2577,.F.);
#22295=ADVANCED_FACE('',(#3514),#21339,.F.);
#22296=ADVANCED_FACE('',(#3515),#2578,.F.);
#22297=ADVANCED_FACE('',(#3516),#21340,.F.);
#22298=ADVANCED_FACE('',(#3517),#2579,.F.);
#22299=ADVANCED_FACE('',(#3518),#21341,.F.);
#22300=ADVANCED_FACE('',(#3519),#2580,.F.);
#22301=ADVANCED_FACE('',(#3520),#21342,.F.);
#22302=ADVANCED_FACE('',(#3521),#2581,.F.);
#22303=ADVANCED_FACE('',(#3522),#21343,.F.);
#22304=ADVANCED_FACE('',(#3523),#2582,.F.);
#22305=ADVANCED_FACE('',(#3524),#21344,.F.);
#22306=ADVANCED_FACE('',(#3525),#2583,.F.);
#22307=ADVANCED_FACE('',(#3526),#21345,.F.);
#22308=ADVANCED_FACE('',(#3527),#2584,.F.);
#22309=ADVANCED_FACE('',(#3528),#21346,.F.);
#22310=ADVANCED_FACE('',(#3529,#2085),#2585,.T.);
#22311=ADVANCED_FACE('',(#3530),#21347,.F.);
#22312=ADVANCED_FACE('',(#3531,#2086),#2586,.T.);
#22313=ADVANCED_FACE('',(#3532),#21348,.F.);
#22314=ADVANCED_FACE('',(#3533,#2087),#2587,.T.);
#22315=ADVANCED_FACE('',(#3534),#21349,.F.);
#22316=ADVANCED_FACE('',(#3535,#2088),#2588,.T.);
#22317=ADVANCED_FACE('',(#3536),#21350,.F.);
#22318=ADVANCED_FACE('',(#3537),#21351,.F.);
#22319=ADVANCED_FACE('',(#3538),#21352,.F.);
#22320=ADVANCED_FACE('',(#3539),#21353,.F.);
#22321=ADVANCED_FACE('',(#3540),#21354,.F.);
#22322=ADVANCED_FACE('',(#3541),#21355,.F.);
#22323=ADVANCED_FACE('',(#3542),#21356,.F.);
#22324=ADVANCED_FACE('',(#3543),#21357,.F.);
#22325=ADVANCED_FACE('',(#3544),#21358,.F.);
#22326=ADVANCED_FACE('',(#3545),#21359,.F.);
#22327=ADVANCED_FACE('',(#3546),#21360,.F.);
#22328=ADVANCED_FACE('',(#3547),#21361,.F.);
#22329=ADVANCED_FACE('',(#3548),#21362,.F.);
#22330=ADVANCED_FACE('',(#3549),#21363,.F.);
#22331=ADVANCED_FACE('',(#3550),#2589,.T.);
#22332=ADVANCED_FACE('',(#3551),#2590,.T.);
#22333=ADVANCED_FACE('',(#3552),#2591,.T.);
#22334=ADVANCED_FACE('',(#3553),#2592,.T.);
#22335=ADVANCED_FACE('',(#3554,#2089,#2090,#2091,#2092,#2093,#2094,#2095,
#2096,#2097,#2098,#2099,#2100,#2101,#2102),#2593,.T.);
#22336=ADVANCED_FACE('',(#3555,#2103,#2104,#2105,#2106,#2107,#2108,#2109,
#2110,#2111,#2112,#2113,#2114,#2115,#2116,#2117,#2118,#2119,#2120,#2121,
#2122,#2123,#2124),#2594,.F.);
#23025=CLOSED_SHELL('',(#22293,#22294,#22295,#22296,#22297,#22298,#22299,
#22300,#22301,#22302,#22303,#22304,#22305,#22306,#22307,#22308,#22309,#22310,
#22311,#22312,#22313,#22314,#22315,#22316,#22317,#22318,#22319,#22320,#22321,
#22322,#22323,#22324,#22325,#22326,#22327,#22328,#22329,#22330,#22331,#22332,
#22333,#22334,#22335,#22336));
#25202=AXIS2_PLACEMENT_3D('',#47781,#29603,#29604);
#25203=AXIS2_PLACEMENT_3D('',#47782,#29605,#29606);
#25204=AXIS2_PLACEMENT_3D('',#47784,#29607,#29608);
#25205=AXIS2_PLACEMENT_3D('',#47787,#29610,#29611);
#25206=AXIS2_PLACEMENT_3D('',#47788,#29612,#29613);
#25207=AXIS2_PLACEMENT_3D('',#47789,#29614,#29615);
#25208=AXIS2_PLACEMENT_3D('',#47791,#29616,#29617);
#25209=AXIS2_PLACEMENT_3D('',#47794,#29619,#29620);
#25210=AXIS2_PLACEMENT_3D('',#47795,#29621,#29622);
#25211=AXIS2_PLACEMENT_3D('',#47796,#29623,#29624);
#25212=AXIS2_PLACEMENT_3D('',#47798,#29625,#29626);
#25213=AXIS2_PLACEMENT_3D('',#47801,#29628,#29629);
#25214=AXIS2_PLACEMENT_3D('',#47802,#29630,#29631);
#25215=AXIS2_PLACEMENT_3D('',#47803,#29632,#29633);
#25216=AXIS2_PLACEMENT_3D('',#47805,#29634,#29635);
#25217=AXIS2_PLACEMENT_3D('',#47808,#29637,#29638);
#25218=AXIS2_PLACEMENT_3D('',#47809,#29639,#29640);
#25219=AXIS2_PLACEMENT_3D('',#47810,#29641,#29642);
#25220=AXIS2_PLACEMENT_3D('',#47812,#29643,#29644);
#25221=AXIS2_PLACEMENT_3D('',#47815,#29646,#29647);
#25222=AXIS2_PLACEMENT_3D('',#47816,#29648,#29649);
#25223=AXIS2_PLACEMENT_3D('',#47817,#29650,#29651);
#25224=AXIS2_PLACEMENT_3D('',#47819,#29652,#29653);
#25225=AXIS2_PLACEMENT_3D('',#47822,#29655,#29656);
#25226=AXIS2_PLACEMENT_3D('',#47823,#29657,#29658);
#25227=AXIS2_PLACEMENT_3D('',#47824,#29659,#29660);
#25228=AXIS2_PLACEMENT_3D('',#47826,#29661,#29662);
#25229=AXIS2_PLACEMENT_3D('',#47829,#29664,#29665);
#25230=AXIS2_PLACEMENT_3D('',#47830,#29666,#29667);
#25231=AXIS2_PLACEMENT_3D('',#47831,#29668,#29669);
#25232=AXIS2_PLACEMENT_3D('',#47833,#29670,#29671);
#25233=AXIS2_PLACEMENT_3D('',#47836,#29673,#29674);
#25234=AXIS2_PLACEMENT_3D('',#47837,#29675,#29676);
#25235=AXIS2_PLACEMENT_3D('',#47838,#29677,#29678);
#25236=AXIS2_PLACEMENT_3D('',#47840,#29679,#29680);
#25237=AXIS2_PLACEMENT_3D('',#47843,#29682,#29683);
#25238=AXIS2_PLACEMENT_3D('',#47844,#29684,#29685);
#25239=AXIS2_PLACEMENT_3D('',#47846,#29686,#29687);
#25240=AXIS2_PLACEMENT_3D('',#47847,#29688,#29689);
#25241=AXIS2_PLACEMENT_3D('',#47849,#29690,#29691);
#25242=AXIS2_PLACEMENT_3D('',#47852,#29693,#29694);
#25243=AXIS2_PLACEMENT_3D('',#47853,#29695,#29696);
#25244=AXIS2_PLACEMENT_3D('',#47855,#29697,#29698);
#25245=AXIS2_PLACEMENT_3D('',#47856,#29699,#29700);
#25246=AXIS2_PLACEMENT_3D('',#47858,#29701,#29702);
#25247=AXIS2_PLACEMENT_3D('',#47861,#29704,#29705);
#25248=AXIS2_PLACEMENT_3D('',#47862,#29706,#29707);
#25249=AXIS2_PLACEMENT_3D('',#47864,#29708,#29709);
#25250=AXIS2_PLACEMENT_3D('',#47865,#29710,#29711);
#25251=AXIS2_PLACEMENT_3D('',#47867,#29712,#29713);
#25252=AXIS2_PLACEMENT_3D('',#47870,#29715,#29716);
#25253=AXIS2_PLACEMENT_3D('',#47871,#29717,#29718);
#25254=AXIS2_PLACEMENT_3D('',#47873,#29719,#29720);
#25255=AXIS2_PLACEMENT_3D('',#47874,#29721,#29722);
#25256=AXIS2_PLACEMENT_3D('',#47876,#29723,#29724);
#25257=AXIS2_PLACEMENT_3D('',#47878,#29726,#29727);
#25258=AXIS2_PLACEMENT_3D('',#47880,#29728,#29729);
#25259=AXIS2_PLACEMENT_3D('',#47882,#29731,#29732);
#25260=AXIS2_PLACEMENT_3D('',#47884,#29733,#29734);
#25261=AXIS2_PLACEMENT_3D('',#47886,#29736,#29737);
#25262=AXIS2_PLACEMENT_3D('',#47888,#29738,#29739);
#25263=AXIS2_PLACEMENT_3D('',#47890,#29741,#29742);
#25264=AXIS2_PLACEMENT_3D('',#47892,#29743,#29744);
#25265=AXIS2_PLACEMENT_3D('',#47895,#29746,#29747);
#25266=AXIS2_PLACEMENT_3D('',#47896,#29748,#29749);
#25267=AXIS2_PLACEMENT_3D('',#47898,#29750,#29751);
#25268=AXIS2_PLACEMENT_3D('',#47901,#29753,#29754);
#25269=AXIS2_PLACEMENT_3D('',#47902,#29755,#29756);
#25270=AXIS2_PLACEMENT_3D('',#47904,#29757,#29758);
#25271=AXIS2_PLACEMENT_3D('',#47907,#29760,#29761);
#25272=AXIS2_PLACEMENT_3D('',#47908,#29762,#29763);
#25273=AXIS2_PLACEMENT_3D('',#47910,#29764,#29765);
#25274=AXIS2_PLACEMENT_3D('',#47913,#29767,#29768);
#25275=AXIS2_PLACEMENT_3D('',#47914,#29769,#29770);
#25276=AXIS2_PLACEMENT_3D('',#47916,#29771,#29772);
#25277=AXIS2_PLACEMENT_3D('',#47919,#29774,#29775);
#25278=AXIS2_PLACEMENT_3D('',#47920,#29776,#29777);
#25279=AXIS2_PLACEMENT_3D('',#47922,#29778,#29779);
#25280=AXIS2_PLACEMENT_3D('',#47925,#29781,#29782);
#25281=AXIS2_PLACEMENT_3D('',#47926,#29783,#29784);
#25282=AXIS2_PLACEMENT_3D('',#47928,#29785,#29786);
#25283=AXIS2_PLACEMENT_3D('',#47931,#29788,#29789);
#25284=AXIS2_PLACEMENT_3D('',#47932,#29790,#29791);
#25285=AXIS2_PLACEMENT_3D('',#47934,#29792,#29793);
#25286=AXIS2_PLACEMENT_3D('',#47937,#29795,#29796);
#25287=AXIS2_PLACEMENT_3D('',#47938,#29797,#29798);
#25288=AXIS2_PLACEMENT_3D('',#47940,#29799,#29800);
#25289=AXIS2_PLACEMENT_3D('',#47943,#29802,#29803);
#25290=AXIS2_PLACEMENT_3D('',#47944,#29804,#29805);
#25291=AXIS2_PLACEMENT_3D('',#47946,#29806,#29807);
#25292=AXIS2_PLACEMENT_3D('',#47949,#29809,#29810);
#25293=AXIS2_PLACEMENT_3D('',#47950,#29811,#29812);
#25294=AXIS2_PLACEMENT_3D('',#47959,#29817,#29818);
#25295=AXIS2_PLACEMENT_3D('',#47965,#29822,#29823);
#25296=AXIS2_PLACEMENT_3D('',#47971,#29827,#29828);
#25297=AXIS2_PLACEMENT_3D('',#47974,#29831,#29832);
#25298=AXIS2_PLACEMENT_3D('',#47975,#29833,#29834);
#29603=DIRECTION('axis',(0.,0.,1.));
#29604=DIRECTION('refdir',(1.,0.,0.));
#29605=DIRECTION('center_axis',(0.,0.,1.));
#29606=DIRECTION('ref_axis',(1.,0.,0.));
#29607=DIRECTION('center_axis',(0.,0.,1.));
#29608=DIRECTION('ref_axis',(1.,0.,0.));
#29609=DIRECTION('',(0.,0.,1.));
#29610=DIRECTION('center_axis',(0.,0.,1.));
#29611=DIRECTION('ref_axis',(1.,0.,0.));
#29612=DIRECTION('center_axis',(0.,0.,1.));
#29613=DIRECTION('ref_axis',(1.,0.,0.));
#29614=DIRECTION('center_axis',(0.,0.,1.));
#29615=DIRECTION('ref_axis',(1.,0.,0.));
#29616=DIRECTION('center_axis',(0.,0.,1.));
#29617=DIRECTION('ref_axis',(1.,0.,0.));
#29618=DIRECTION('',(0.,0.,1.));
#29619=DIRECTION('center_axis',(0.,0.,1.));
#29620=DIRECTION('ref_axis',(1.,0.,0.));
#29621=DIRECTION('center_axis',(0.,0.,1.));
#29622=DIRECTION('ref_axis',(1.,0.,0.));
#29623=DIRECTION('center_axis',(0.,0.,1.));
#29624=DIRECTION('ref_axis',(1.,0.,0.));
#29625=DIRECTION('center_axis',(0.,0.,1.));
#29626=DIRECTION('ref_axis',(1.,0.,0.));
#29627=DIRECTION('',(0.,0.,1.));
#29628=DIRECTION('center_axis',(0.,0.,1.));
#29629=DIRECTION('ref_axis',(1.,0.,0.));
#29630=DIRECTION('center_axis',(0.,0.,1.));
#29631=DIRECTION('ref_axis',(1.,0.,0.));
#29632=DIRECTION('center_axis',(0.,0.,1.));
#29633=DIRECTION('ref_axis',(1.,0.,0.));
#29634=DIRECTION('center_axis',(0.,0.,1.));
#29635=DIRECTION('ref_axis',(1.,0.,0.));
#29636=DIRECTION('',(0.,0.,1.));
#29637=DIRECTION('center_axis',(0.,0.,1.));
#29638=DIRECTION('ref_axis',(1.,0.,0.));
#29639=DIRECTION('center_axis',(0.,0.,1.));
#29640=DIRECTION('ref_axis',(1.,0.,0.));
#29641=DIRECTION('center_axis',(0.,0.,1.));
#29642=DIRECTION('ref_axis',(1.,0.,0.));
#29643=DIRECTION('center_axis',(0.,0.,1.));
#29644=DIRECTION('ref_axis',(1.,0.,0.));
#29645=DIRECTION('',(0.,0.,1.));
#29646=DIRECTION('center_axis',(0.,0.,1.));
#29647=DIRECTION('ref_axis',(1.,0.,0.));
#29648=DIRECTION('center_axis',(0.,0.,1.));
#29649=DIRECTION('ref_axis',(1.,0.,0.));
#29650=DIRECTION('center_axis',(0.,0.,1.));
#29651=DIRECTION('ref_axis',(1.,0.,0.));
#29652=DIRECTION('center_axis',(0.,0.,1.));
#29653=DIRECTION('ref_axis',(1.,0.,0.));
#29654=DIRECTION('',(0.,0.,1.));
#29655=DIRECTION('center_axis',(0.,0.,1.));
#29656=DIRECTION('ref_axis',(1.,0.,0.));
#29657=DIRECTION('center_axis',(0.,0.,1.));
#29658=DIRECTION('ref_axis',(1.,0.,0.));
#29659=DIRECTION('center_axis',(0.,0.,1.));
#29660=DIRECTION('ref_axis',(1.,0.,0.));
#29661=DIRECTION('center_axis',(0.,0.,1.));
#29662=DIRECTION('ref_axis',(1.,0.,0.));
#29663=DIRECTION('',(0.,0.,1.));
#29664=DIRECTION('center_axis',(0.,0.,1.));
#29665=DIRECTION('ref_axis',(1.,0.,0.));
#29666=DIRECTION('center_axis',(0.,0.,1.));
#29667=DIRECTION('ref_axis',(1.,0.,0.));
#29668=DIRECTION('center_axis',(0.,0.,1.));
#29669=DIRECTION('ref_axis',(1.,0.,0.));
#29670=DIRECTION('center_axis',(0.,0.,1.));
#29671=DIRECTION('ref_axis',(1.,0.,0.));
#29672=DIRECTION('',(0.,0.,1.));
#29673=DIRECTION('center_axis',(0.,0.,1.));
#29674=DIRECTION('ref_axis',(1.,0.,0.));
#29675=DIRECTION('center_axis',(0.,0.,1.));
#29676=DIRECTION('ref_axis',(1.,0.,0.));
#29677=DIRECTION('center_axis',(0.,0.,1.));
#29678=DIRECTION('ref_axis',(1.,0.,0.));
#29679=DIRECTION('center_axis',(0.,0.,1.));
#29680=DIRECTION('ref_axis',(1.,0.,0.));
#29681=DIRECTION('',(0.,0.,1.));
#29682=DIRECTION('center_axis',(0.,0.,-1.));
#29683=DIRECTION('ref_axis',(1.,0.,0.));
#29684=DIRECTION('center_axis',(0.,0.,1.));
#29685=DIRECTION('ref_axis',(1.,0.,0.));
#29686=DIRECTION('center_axis',(0.,0.,1.));
#29687=DIRECTION('ref_axis',(1.,0.,0.));
#29688=DIRECTION('center_axis',(0.,0.,1.));
#29689=DIRECTION('ref_axis',(1.,0.,0.));
#29690=DIRECTION('center_axis',(0.,0.,1.));
#29691=DIRECTION('ref_axis',(1.,0.,0.));
#29692=DIRECTION('',(0.,0.,1.));
#29693=DIRECTION('center_axis',(0.,0.,-1.));
#29694=DIRECTION('ref_axis',(1.,0.,0.));
#29695=DIRECTION('center_axis',(0.,0.,1.));
#29696=DIRECTION('ref_axis',(1.,0.,0.));
#29697=DIRECTION('center_axis',(0.,0.,1.));
#29698=DIRECTION('ref_axis',(1.,0.,0.));
#29699=DIRECTION('center_axis',(0.,0.,1.));
#29700=DIRECTION('ref_axis',(1.,0.,0.));
#29701=DIRECTION('center_axis',(0.,0.,1.));
#29702=DIRECTION('ref_axis',(1.,0.,0.));
#29703=DIRECTION('',(0.,0.,1.));
#29704=DIRECTION('center_axis',(0.,0.,-1.));
#29705=DIRECTION('ref_axis',(1.,0.,0.));
#29706=DIRECTION('center_axis',(0.,0.,1.));
#29707=DIRECTION('ref_axis',(1.,0.,0.));
#29708=DIRECTION('center_axis',(0.,0.,1.));
#29709=DIRECTION('ref_axis',(1.,0.,0.));
#29710=DIRECTION('center_axis',(0.,0.,1.));
#29711=DIRECTION('ref_axis',(1.,0.,0.));
#29712=DIRECTION('center_axis',(0.,0.,1.));
#29713=DIRECTION('ref_axis',(1.,0.,0.));
#29714=DIRECTION('',(0.,0.,1.));
#29715=DIRECTION('center_axis',(0.,0.,-1.));
#29716=DIRECTION('ref_axis',(1.,0.,0.));
#29717=DIRECTION('center_axis',(0.,0.,1.));
#29718=DIRECTION('ref_axis',(1.,0.,0.));
#29719=DIRECTION('center_axis',(0.,0.,1.));
#29720=DIRECTION('ref_axis',(1.,0.,0.));
#29721=DIRECTION('center_axis',(0.,0.,1.));
#29722=DIRECTION('ref_axis',(1.,0.,0.));
#29723=DIRECTION('center_axis',(0.,0.,1.));
#29724=DIRECTION('ref_axis',(1.,0.,0.));
#29725=DIRECTION('',(0.,0.,1.));
#29726=DIRECTION('center_axis',(0.,0.,1.));
#29727=DIRECTION('ref_axis',(1.,0.,0.));
#29728=DIRECTION('center_axis',(0.,0.,1.));
#29729=DIRECTION('ref_axis',(1.,0.,0.));
#29730=DIRECTION('',(0.,0.,1.));
#29731=DIRECTION('center_axis',(0.,0.,1.));
#29732=DIRECTION('ref_axis',(1.,0.,0.));
#29733=DIRECTION('center_axis',(0.,0.,1.));
#29734=DIRECTION('ref_axis',(1.,0.,0.));
#29735=DIRECTION('',(0.,0.,1.));
#29736=DIRECTION('center_axis',(0.,0.,1.));
#29737=DIRECTION('ref_axis',(1.,0.,0.));
#29738=DIRECTION('center_axis',(0.,0.,1.));
#29739=DIRECTION('ref_axis',(1.,0.,0.));
#29740=DIRECTION('',(0.,0.,1.));
#29741=DIRECTION('center_axis',(0.,0.,1.));
#29742=DIRECTION('ref_axis',(1.,0.,0.));
#29743=DIRECTION('center_axis',(0.,0.,1.));
#29744=DIRECTION('ref_axis',(1.,0.,0.));
#29745=DIRECTION('',(0.,0.,1.));
#29746=DIRECTION('center_axis',(0.,0.,-1.));
#29747=DIRECTION('ref_axis',(1.,0.,0.));
#29748=DIRECTION('center_axis',(0.,0.,1.));
#29749=DIRECTION('ref_axis',(1.,0.,0.));
#29750=DIRECTION('center_axis',(0.,0.,1.));
#29751=DIRECTION('ref_axis',(1.,0.,0.));
#29752=DIRECTION('',(0.,0.,1.));
#29753=DIRECTION('center_axis',(0.,0.,-1.));
#29754=DIRECTION('ref_axis',(1.,0.,0.));
#29755=DIRECTION('center_axis',(0.,0.,1.));
#29756=DIRECTION('ref_axis',(1.,0.,0.));
#29757=DIRECTION('center_axis',(0.,0.,1.));
#29758=DIRECTION('ref_axis',(1.,0.,0.));
#29759=DIRECTION('',(0.,0.,1.));
#29760=DIRECTION('center_axis',(0.,0.,-1.));
#29761=DIRECTION('ref_axis',(1.,0.,0.));
#29762=DIRECTION('center_axis',(0.,0.,1.));
#29763=DIRECTION('ref_axis',(1.,0.,0.));
#29764=DIRECTION('center_axis',(0.,0.,1.));
#29765=DIRECTION('ref_axis',(1.,0.,0.));
#29766=DIRECTION('',(0.,0.,1.));
#29767=DIRECTION('center_axis',(0.,0.,-1.));
#29768=DIRECTION('ref_axis',(1.,0.,0.));
#29769=DIRECTION('center_axis',(0.,0.,1.));
#29770=DIRECTION('ref_axis',(1.,0.,0.));
#29771=DIRECTION('center_axis',(0.,0.,1.));
#29772=DIRECTION('ref_axis',(1.,0.,0.));
#29773=DIRECTION('',(0.,0.,1.));
#29774=DIRECTION('center_axis',(0.,0.,-1.));
#29775=DIRECTION('ref_axis',(1.,0.,0.));
#29776=DIRECTION('center_axis',(0.,0.,1.));
#29777=DIRECTION('ref_axis',(1.,0.,0.));
#29778=DIRECTION('center_axis',(0.,0.,1.));
#29779=DIRECTION('ref_axis',(1.,0.,0.));
#29780=DIRECTION('',(0.,0.,1.));
#29781=DIRECTION('center_axis',(0.,0.,-1.));
#29782=DIRECTION('ref_axis',(1.,0.,0.));
#29783=DIRECTION('center_axis',(0.,0.,1.));
#29784=DIRECTION('ref_axis',(1.,0.,0.));
#29785=DIRECTION('center_axis',(0.,0.,1.));
#29786=DIRECTION('ref_axis',(1.,0.,0.));
#29787=DIRECTION('',(0.,0.,1.));
#29788=DIRECTION('center_axis',(0.,0.,-1.));
#29789=DIRECTION('ref_axis',(1.,0.,0.));
#29790=DIRECTION('center_axis',(0.,0.,1.));
#29791=DIRECTION('ref_axis',(1.,0.,0.));
#29792=DIRECTION('center_axis',(0.,0.,1.));
#29793=DIRECTION('ref_axis',(1.,0.,0.));
#29794=DIRECTION('',(0.,0.,1.));
#29795=DIRECTION('center_axis',(0.,0.,-1.));
#29796=DIRECTION('ref_axis',(1.,0.,0.));
#29797=DIRECTION('center_axis',(0.,0.,1.));
#29798=DIRECTION('ref_axis',(1.,0.,0.));
#29799=DIRECTION('center_axis',(0.,0.,1.));
#29800=DIRECTION('ref_axis',(1.,0.,0.));
#29801=DIRECTION('',(0.,0.,1.));
#29802=DIRECTION('center_axis',(0.,0.,-1.));
#29803=DIRECTION('ref_axis',(1.,0.,0.));
#29804=DIRECTION('center_axis',(0.,0.,1.));
#29805=DIRECTION('ref_axis',(1.,0.,0.));
#29806=DIRECTION('center_axis',(0.,0.,1.));
#29807=DIRECTION('ref_axis',(1.,0.,0.));
#29808=DIRECTION('',(0.,0.,1.));
#29809=DIRECTION('center_axis',(0.,0.,-1.));
#29810=DIRECTION('ref_axis',(1.,0.,0.));
#29811=DIRECTION('center_axis',(0.,1.,0.));
#29812=DIRECTION('ref_axis',(-1.,0.,0.));
#29813=DIRECTION('',(-1.,0.,0.));
#29814=DIRECTION('',(0.,0.,1.));
#29815=DIRECTION('',(-1.,0.,0.));
#29816=DIRECTION('',(0.,0.,1.));
#29817=DIRECTION('center_axis',(1.,0.,0.));
#29818=DIRECTION('ref_axis',(0.,1.,0.));
#29819=DIRECTION('',(0.,1.,0.));
#29820=DIRECTION('',(0.,1.,0.));
#29821=DIRECTION('',(0.,0.,1.));
#29822=DIRECTION('center_axis',(0.,-1.,0.));
#29823=DIRECTION('ref_axis',(1.,0.,0.));
#29824=DIRECTION('',(1.,0.,0.));
#29825=DIRECTION('',(1.,0.,0.));
#29826=DIRECTION('',(0.,0.,1.));
#29827=DIRECTION('center_axis',(-1.,0.,0.));
#29828=DIRECTION('ref_axis',(0.,-1.,0.));
#29829=DIRECTION('',(0.,-1.,0.));
#29830=DIRECTION('',(0.,-1.,0.));
#29831=DIRECTION('center_axis',(0.,0.,1.));
#29832=DIRECTION('ref_axis',(1.,0.,0.));
#29833=DIRECTION('center_axis',(0.,0.,1.));
#29834=DIRECTION('ref_axis',(1.,0.,0.));
#47781=CARTESIAN_POINT('',(0.,0.,0.));
#47782=CARTESIAN_POINT('Origin',(15.5,-5.,-0.1));
#47783=CARTESIAN_POINT('',(14.95,-5.,0.));
#47784=CARTESIAN_POINT('Origin',(15.5,-5.,0.));
#47785=CARTESIAN_POINT('',(14.95,-5.,0.8));
#47786=CARTESIAN_POINT('',(14.95,-5.,-0.1));
#47787=CARTESIAN_POINT('Origin',(15.5,-5.,0.8));
#47788=CARTESIAN_POINT('Origin',(15.5,-5.,0.8));
#47789=CARTESIAN_POINT('Origin',(15.5,-3.5,-0.1));
#47790=CARTESIAN_POINT('',(14.95,-3.5,0.));
#47791=CARTESIAN_POINT('Origin',(15.5,-3.5,0.));
#47792=CARTESIAN_POINT('',(14.95,-3.5,0.8));
#47793=CARTESIAN_POINT('',(14.95,-3.5,-0.1));
#47794=CARTESIAN_POINT('Origin',(15.5,-3.5,0.8));
#47795=CARTESIAN_POINT('Origin',(15.5,-3.5,0.8));
#47796=CARTESIAN_POINT('Origin',(12.9,-6.,-0.1));
#47797=CARTESIAN_POINT('',(12.35,-6.,0.));
#47798=CARTESIAN_POINT('Origin',(12.9,-6.,0.));
#47799=CARTESIAN_POINT('',(12.35,-6.,0.8));
#47800=CARTESIAN_POINT('',(12.35,-6.,-0.1));
#47801=CARTESIAN_POINT('Origin',(12.9,-6.,0.8));
#47802=CARTESIAN_POINT('Origin',(12.9,-6.,0.8));
#47803=CARTESIAN_POINT('Origin',(12.9,-3.,-0.1));
#47804=CARTESIAN_POINT('',(12.35,-3.,0.));
#47805=CARTESIAN_POINT('Origin',(12.9,-3.,0.));
#47806=CARTESIAN_POINT('',(12.35,-3.,0.8));
#47807=CARTESIAN_POINT('',(12.35,-3.,-0.1));
#47808=CARTESIAN_POINT('Origin',(12.9,-3.,0.8));
#47809=CARTESIAN_POINT('Origin',(12.9,-3.,0.8));
#47810=CARTESIAN_POINT('Origin',(9.1,-6.,-0.1));
#47811=CARTESIAN_POINT('',(8.55,-6.,0.));
#47812=CARTESIAN_POINT('Origin',(9.1,-6.,0.));
#47813=CARTESIAN_POINT('',(8.55,-6.,0.8));
#47814=CARTESIAN_POINT('',(8.55,-6.,-0.1));
#47815=CARTESIAN_POINT('Origin',(9.1,-6.,0.8));
#47816=CARTESIAN_POINT('Origin',(9.1,-6.,0.8));
#47817=CARTESIAN_POINT('Origin',(9.1,-3.,-0.1));
#47818=CARTESIAN_POINT('',(8.55,-3.,0.));
#47819=CARTESIAN_POINT('Origin',(9.1,-3.,0.));
#47820=CARTESIAN_POINT('',(8.55,-3.,0.8));
#47821=CARTESIAN_POINT('',(8.55,-3.,-0.1));
#47822=CARTESIAN_POINT('Origin',(9.1,-3.,0.8));
#47823=CARTESIAN_POINT('Origin',(9.1,-3.,0.8));
#47824=CARTESIAN_POINT('Origin',(18.5,-3.5,-0.1));
#47825=CARTESIAN_POINT('',(17.95,-3.5,0.));
#47826=CARTESIAN_POINT('Origin',(18.5,-3.5,0.));
#47827=CARTESIAN_POINT('',(17.95,-3.5,0.8));
#47828=CARTESIAN_POINT('',(17.95,-3.5,-0.1));
#47829=CARTESIAN_POINT('Origin',(18.5,-3.5,0.8));
#47830=CARTESIAN_POINT('Origin',(18.5,-3.5,0.8));
#47831=CARTESIAN_POINT('Origin',(18.5,-5.,-0.1));
#47832=CARTESIAN_POINT('',(17.95,-5.,0.));
#47833=CARTESIAN_POINT('Origin',(18.5,-5.,0.));
#47834=CARTESIAN_POINT('',(17.95,-5.,0.8));
#47835=CARTESIAN_POINT('',(17.95,-5.,-0.1));
#47836=CARTESIAN_POINT('Origin',(18.5,-5.,0.8));
#47837=CARTESIAN_POINT('Origin',(18.5,-5.,0.8));
#47838=CARTESIAN_POINT('Origin',(8.,-7.2,0.6));
#47839=CARTESIAN_POINT('',(7.5,-7.2,0.6));
#47840=CARTESIAN_POINT('Origin',(8.,-7.2,0.6));
#47841=CARTESIAN_POINT('',(7.5,-7.2,1.2));
#47842=CARTESIAN_POINT('',(7.5,-7.2,0.6));
#47843=CARTESIAN_POINT('Origin',(8.,-7.2,1.2));
#47844=CARTESIAN_POINT('Origin',(8.,-7.2,0.6));
#47845=CARTESIAN_POINT('',(7.725,-7.2,0.6));
#47846=CARTESIAN_POINT('Origin',(8.,-7.2,0.6));
#47847=CARTESIAN_POINT('Origin',(18.,-1.8,0.6));
#47848=CARTESIAN_POINT('',(17.5,-1.8,0.6));
#47849=CARTESIAN_POINT('Origin',(18.,-1.8,0.6));
#47850=CARTESIAN_POINT('',(17.5,-1.8,1.2));
#47851=CARTESIAN_POINT('',(17.5,-1.8,0.6));
#47852=CARTESIAN_POINT('Origin',(18.,-1.8,1.2));
#47853=CARTESIAN_POINT('Origin',(18.,-1.8,0.6));
#47854=CARTESIAN_POINT('',(17.725,-1.8,0.6));
#47855=CARTESIAN_POINT('Origin',(18.,-1.8,0.6));
#47856=CARTESIAN_POINT('Origin',(8.,-1.8,0.6));
#47857=CARTESIAN_POINT('',(7.5,-1.8,0.6));
#47858=CARTESIAN_POINT('Origin',(8.,-1.8,0.6));
#47859=CARTESIAN_POINT('',(7.5,-1.8,1.2));
#47860=CARTESIAN_POINT('',(7.5,-1.8,0.6));
#47861=CARTESIAN_POINT('Origin',(8.,-1.8,1.2));
#47862=CARTESIAN_POINT('Origin',(8.,-1.8,0.6));
#47863=CARTESIAN_POINT('',(7.725,-1.8,0.6));
#47864=CARTESIAN_POINT('Origin',(8.,-1.8,0.6));
#47865=CARTESIAN_POINT('Origin',(18.,-7.2,0.6));
#47866=CARTESIAN_POINT('',(17.5,-7.2,0.6));
#47867=CARTESIAN_POINT('Origin',(18.,-7.2,0.6));
#47868=CARTESIAN_POINT('',(17.5,-7.2,1.2));
#47869=CARTESIAN_POINT('',(17.5,-7.2,0.6));
#47870=CARTESIAN_POINT('Origin',(18.,-7.2,1.2));
#47871=CARTESIAN_POINT('Origin',(18.,-7.2,0.6));
#47872=CARTESIAN_POINT('',(17.725,-7.2,0.6));
#47873=CARTESIAN_POINT('Origin',(18.,-7.2,0.6));
#47874=CARTESIAN_POINT('Origin',(8.,-7.2,-0.1));
#47875=CARTESIAN_POINT('',(7.725,-7.2,0.));
#47876=CARTESIAN_POINT('Origin',(8.,-7.2,0.));
#47877=CARTESIAN_POINT('',(7.725,-7.2,-0.1));
#47878=CARTESIAN_POINT('Origin',(18.,-1.8,-0.1));
#47879=CARTESIAN_POINT('',(17.725,-1.8,0.));
#47880=CARTESIAN_POINT('Origin',(18.,-1.8,0.));
#47881=CARTESIAN_POINT('',(17.725,-1.8,-0.1));
#47882=CARTESIAN_POINT('Origin',(8.,-1.8,-0.1));
#47883=CARTESIAN_POINT('',(7.725,-1.8,0.));
#47884=CARTESIAN_POINT('Origin',(8.,-1.8,0.));
#47885=CARTESIAN_POINT('',(7.725,-1.8,-0.1));
#47886=CARTESIAN_POINT('Origin',(18.,-7.2,-0.1));
#47887=CARTESIAN_POINT('',(17.725,-7.2,0.));
#47888=CARTESIAN_POINT('Origin',(18.,-7.2,0.));
#47889=CARTESIAN_POINT('',(17.725,-7.2,-0.1));
#47890=CARTESIAN_POINT('Origin',(23.5,-9.25,-0.1));
#47891=CARTESIAN_POINT('',(23.29,-9.25,0.));
#47892=CARTESIAN_POINT('Origin',(23.5,-9.25,0.));
#47893=CARTESIAN_POINT('',(23.29,-9.25,1.2));
#47894=CARTESIAN_POINT('',(23.29,-9.25,-0.1));
#47895=CARTESIAN_POINT('Origin',(23.5,-9.25,1.2));
#47896=CARTESIAN_POINT('Origin',(3.5,-9.25,-0.1));
#47897=CARTESIAN_POINT('',(3.29,-9.25,0.));
#47898=CARTESIAN_POINT('Origin',(3.5,-9.25,0.));
#47899=CARTESIAN_POINT('',(3.29,-9.25,1.2));
#47900=CARTESIAN_POINT('',(3.29,-9.25,-0.1));
#47901=CARTESIAN_POINT('Origin',(3.5,-9.25,1.2));
#47902=CARTESIAN_POINT('Origin',(24.,-3.5,-0.1));
#47903=CARTESIAN_POINT('',(23.67,-3.5,0.));
#47904=CARTESIAN_POINT('Origin',(24.,-3.5,0.));
#47905=CARTESIAN_POINT('',(23.67,-3.5,1.2));
#47906=CARTESIAN_POINT('',(23.67,-3.5,-0.1));
#47907=CARTESIAN_POINT('Origin',(24.,-3.5,1.2));
#47908=CARTESIAN_POINT('Origin',(24.,3.5,-0.1));
#47909=CARTESIAN_POINT('',(23.67,3.5,0.));
#47910=CARTESIAN_POINT('Origin',(24.,3.5,0.));
#47911=CARTESIAN_POINT('',(23.67,3.5,1.2));
#47912=CARTESIAN_POINT('',(23.67,3.5,-0.1));
#47913=CARTESIAN_POINT('Origin',(24.,3.5,1.2));
#47914=CARTESIAN_POINT('Origin',(3.,-2.4,-0.1));
#47915=CARTESIAN_POINT('',(2.725,-2.4,0.));
#47916=CARTESIAN_POINT('Origin',(3.,-2.4,0.));
#47917=CARTESIAN_POINT('',(2.725,-2.4,1.2));
#47918=CARTESIAN_POINT('',(2.725,-2.4,-0.1));
#47919=CARTESIAN_POINT('Origin',(3.,-2.4,1.2));
#47920=CARTESIAN_POINT('Origin',(3.,2.4,-0.1));
#47921=CARTESIAN_POINT('',(2.725,2.4,0.));
#47922=CARTESIAN_POINT('Origin',(3.,2.4,0.));
#47923=CARTESIAN_POINT('',(2.725,2.4,1.2));
#47924=CARTESIAN_POINT('',(2.725,2.4,-0.1));
#47925=CARTESIAN_POINT('Origin',(3.,2.4,1.2));
#47926=CARTESIAN_POINT('Origin',(26.,-7.8,-0.1));
#47927=CARTESIAN_POINT('',(25.79,-7.8,0.));
#47928=CARTESIAN_POINT('Origin',(26.,-7.8,0.));
#47929=CARTESIAN_POINT('',(25.79,-7.8,1.2));
#47930=CARTESIAN_POINT('',(25.79,-7.8,-0.1));
#47931=CARTESIAN_POINT('Origin',(26.,-7.8,1.2));
#47932=CARTESIAN_POINT('Origin',(1.,-5.5,-0.1));
#47933=CARTESIAN_POINT('',(0.79,-5.5,0.));
#47934=CARTESIAN_POINT('Origin',(1.,-5.5,0.));
#47935=CARTESIAN_POINT('',(0.79,-5.5,1.2));
#47936=CARTESIAN_POINT('',(0.79,-5.5,-0.1));
#47937=CARTESIAN_POINT('Origin',(1.,-5.5,1.2));
#47938=CARTESIAN_POINT('Origin',(1.,-7.8,-0.1));
#47939=CARTESIAN_POINT('',(0.79,-7.8,0.));
#47940=CARTESIAN_POINT('Origin',(1.,-7.8,0.));
#47941=CARTESIAN_POINT('',(0.79,-7.8,1.2));
#47942=CARTESIAN_POINT('',(0.79,-7.8,-0.1));
#47943=CARTESIAN_POINT('Origin',(1.,-7.8,1.2));
#47944=CARTESIAN_POINT('Origin',(26.,-5.5,-0.1));
#47945=CARTESIAN_POINT('',(25.79,-5.5,0.));
#47946=CARTESIAN_POINT('Origin',(26.,-5.5,0.));
#47947=CARTESIAN_POINT('',(25.79,-5.5,1.2));
#47948=CARTESIAN_POINT('',(25.79,-5.5,-0.1));
#47949=CARTESIAN_POINT('Origin',(26.,-5.5,1.2));
#47950=CARTESIAN_POINT('Origin',(27.,5.,0.));
#47951=CARTESIAN_POINT('',(27.,5.,0.));
#47952=CARTESIAN_POINT('',(0.,5.,0.));
#47953=CARTESIAN_POINT('',(27.,5.,0.));
#47954=CARTESIAN_POINT('',(0.,5.,1.2));
#47955=CARTESIAN_POINT('',(0.,5.,0.));
#47956=CARTESIAN_POINT('',(27.,5.,1.2));
#47957=CARTESIAN_POINT('',(27.,5.,1.2));
#47958=CARTESIAN_POINT('',(27.,5.,0.));
#47959=CARTESIAN_POINT('Origin',(27.,-10.,0.));
#47960=CARTESIAN_POINT('',(27.,-10.,0.));
#47961=CARTESIAN_POINT('',(27.,-10.,0.));
#47962=CARTESIAN_POINT('',(27.,-10.,1.2));
#47963=CARTESIAN_POINT('',(27.,-10.,1.2));
#47964=CARTESIAN_POINT('',(27.,-10.,0.));
#47965=CARTESIAN_POINT('Origin',(0.,-10.,0.));
#47966=CARTESIAN_POINT('',(0.,-10.,0.));
#47967=CARTESIAN_POINT('',(0.,-10.,0.));
#47968=CARTESIAN_POINT('',(0.,-10.,1.2));
#47969=CARTESIAN_POINT('',(0.,-10.,1.2));
#47970=CARTESIAN_POINT('',(0.,-10.,0.));
#47971=CARTESIAN_POINT('Origin',(0.,5.,0.));
#47972=CARTESIAN_POINT('',(0.,5.,0.));
#47973=CARTESIAN_POINT('',(0.,5.,1.2));
#47974=CARTESIAN_POINT('Origin',(13.5,-2.5,1.2));
#47975=CARTESIAN_POINT('Origin',(13.5,-2.5,0.));
#62839=UNCERTAINTY_MEASURE_WITH_UNIT(LENGTH_MEASURE(0.001),#62985,
'DISTANCE_ACCURACY_VALUE',
'Maximum model space distance between geometric entities at asserted c
onnectivities');
#62885=UNCERTAINTY_MEASURE_WITH_UNIT(LENGTH_MEASURE(0.001),#62985,
'DISTANCE_ACCURACY_VALUE',
'Maximum model space distance between geometric entities at asserted c
onnectivities');
#62938=(
GEOMETRIC_REPRESENTATION_CONTEXT(3)
GLOBAL_UNCERTAINTY_ASSIGNED_CONTEXT((#62839))
GLOBAL_UNIT_ASSIGNED_CONTEXT((#62985,#62987,#62988))
REPRESENTATION_CONTEXT('','3D')
);
#62984=(
GEOMETRIC_REPRESENTATION_CONTEXT(3)
GLOBAL_UNCERTAINTY_ASSIGNED_CONTEXT((#62885))
GLOBAL_UNIT_ASSIGNED_CONTEXT((#62985,#62987,#62988))
REPRESENTATION_CONTEXT('','3D')
);
#62985=(
LENGTH_UNIT()
NAMED_UNIT(*)
SI_UNIT(.CENTI.,.METRE.)
);
#62987=(
NAMED_UNIT(*)
PLANE_ANGLE_UNIT()
SI_UNIT($,.RADIAN.)
);
#62988=(
NAMED_UNIT(*)
SI_UNIT($,.STERADIAN.)
SOLID_ANGLE_UNIT()
);
#63041=SHAPE_DEFINITION_REPRESENTATION(#63219,#63401);
#63219=PRODUCT_DEFINITION_SHAPE('',$,#63500);
#63401=SHAPE_REPRESENTATION('',(#25202),#62938);
#63447=PRODUCT_DEFINITION_CONTEXT('part definition',#63743,'design');
#63500=PRODUCT_DEFINITION('Y Stage - 02 Base','Y Stage - 02 Base',#63598,
#63447);
#63598=PRODUCT_DEFINITION_FORMATION('',$,#63797);
#63743=APPLICATION_CONTEXT(
'Core Data for Automotive Mechanical Design Process');
#63744=PRODUCT_CONTEXT('part definition',#63743,'mechanical');
#63797=PRODUCT('Y Stage - 02 Base','Y Stage - 02 Base',
'Y Stage - 02 Base',(#63744));
#63885=COLOUR_RGB('Dark Blue',0.08,0.2,0.34);
#63886=FILL_AREA_STYLE_COLOUR('',#63885);
#63887=FILL_AREA_STYLE('',(#63886));
#63888=SURFACE_STYLE_FILL_AREA(#63887);
#63889=SURFACE_SIDE_STYLE('',(#63888));
#63890=SURFACE_STYLE_USAGE(.BOTH.,#63889);
#63891=PRESENTATION_STYLE_ASSIGNMENT((#63890));
ENDSEC;
END-ISO-10303-21;
